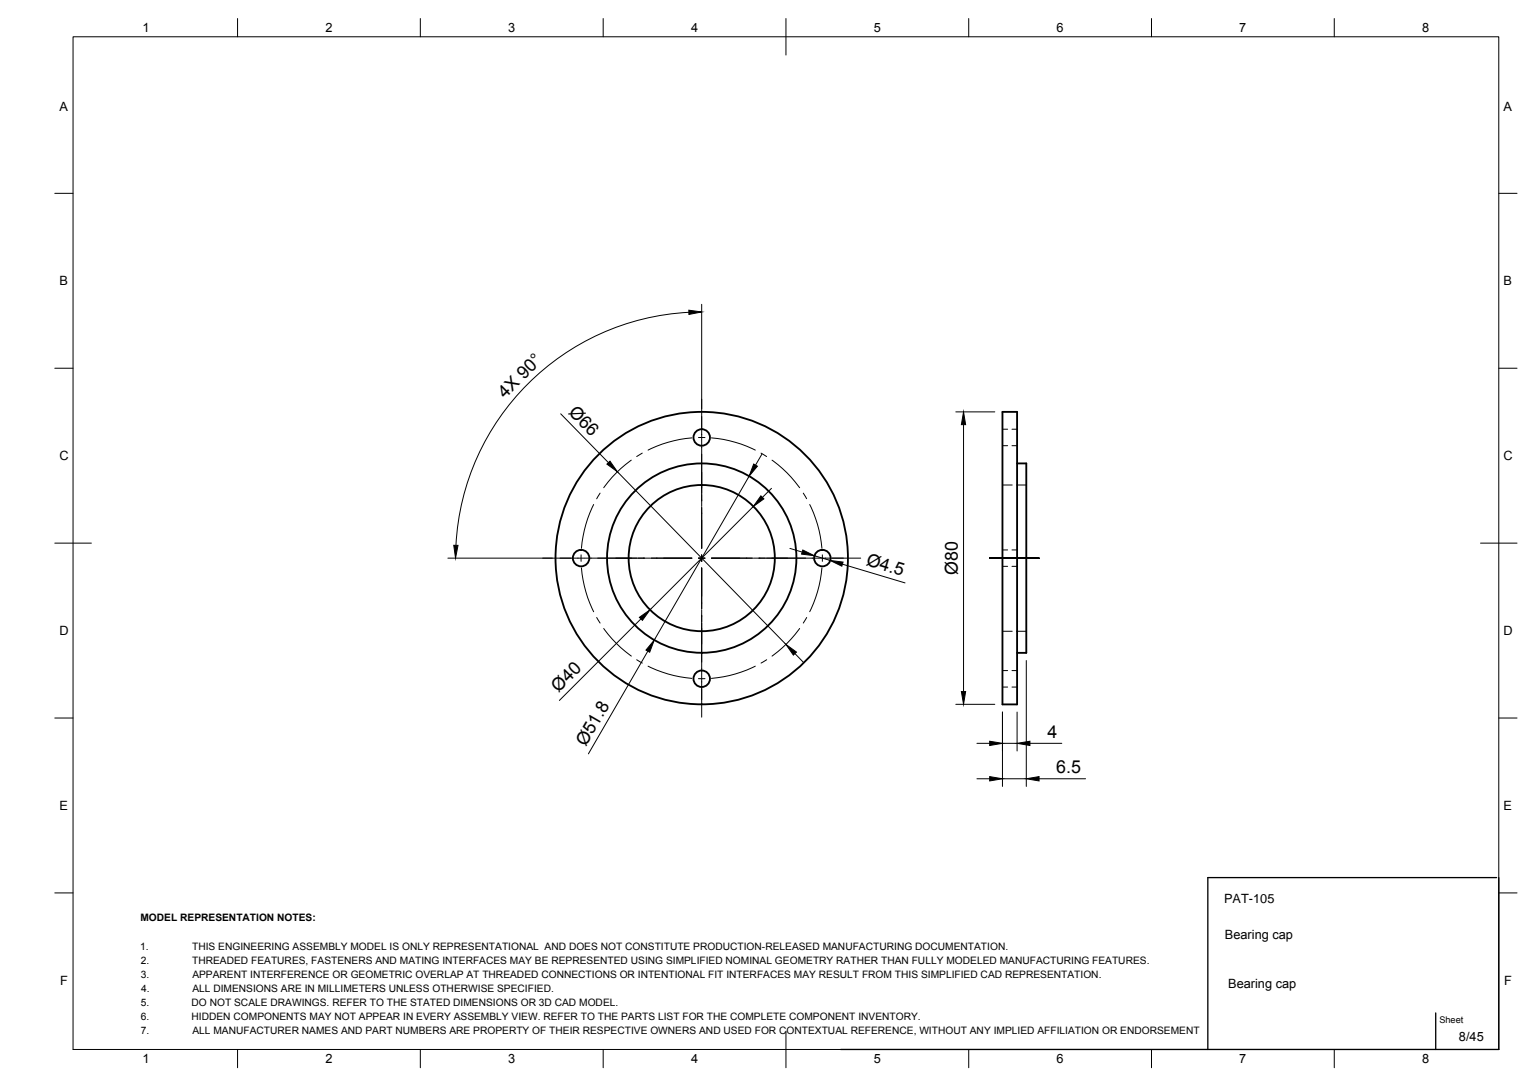
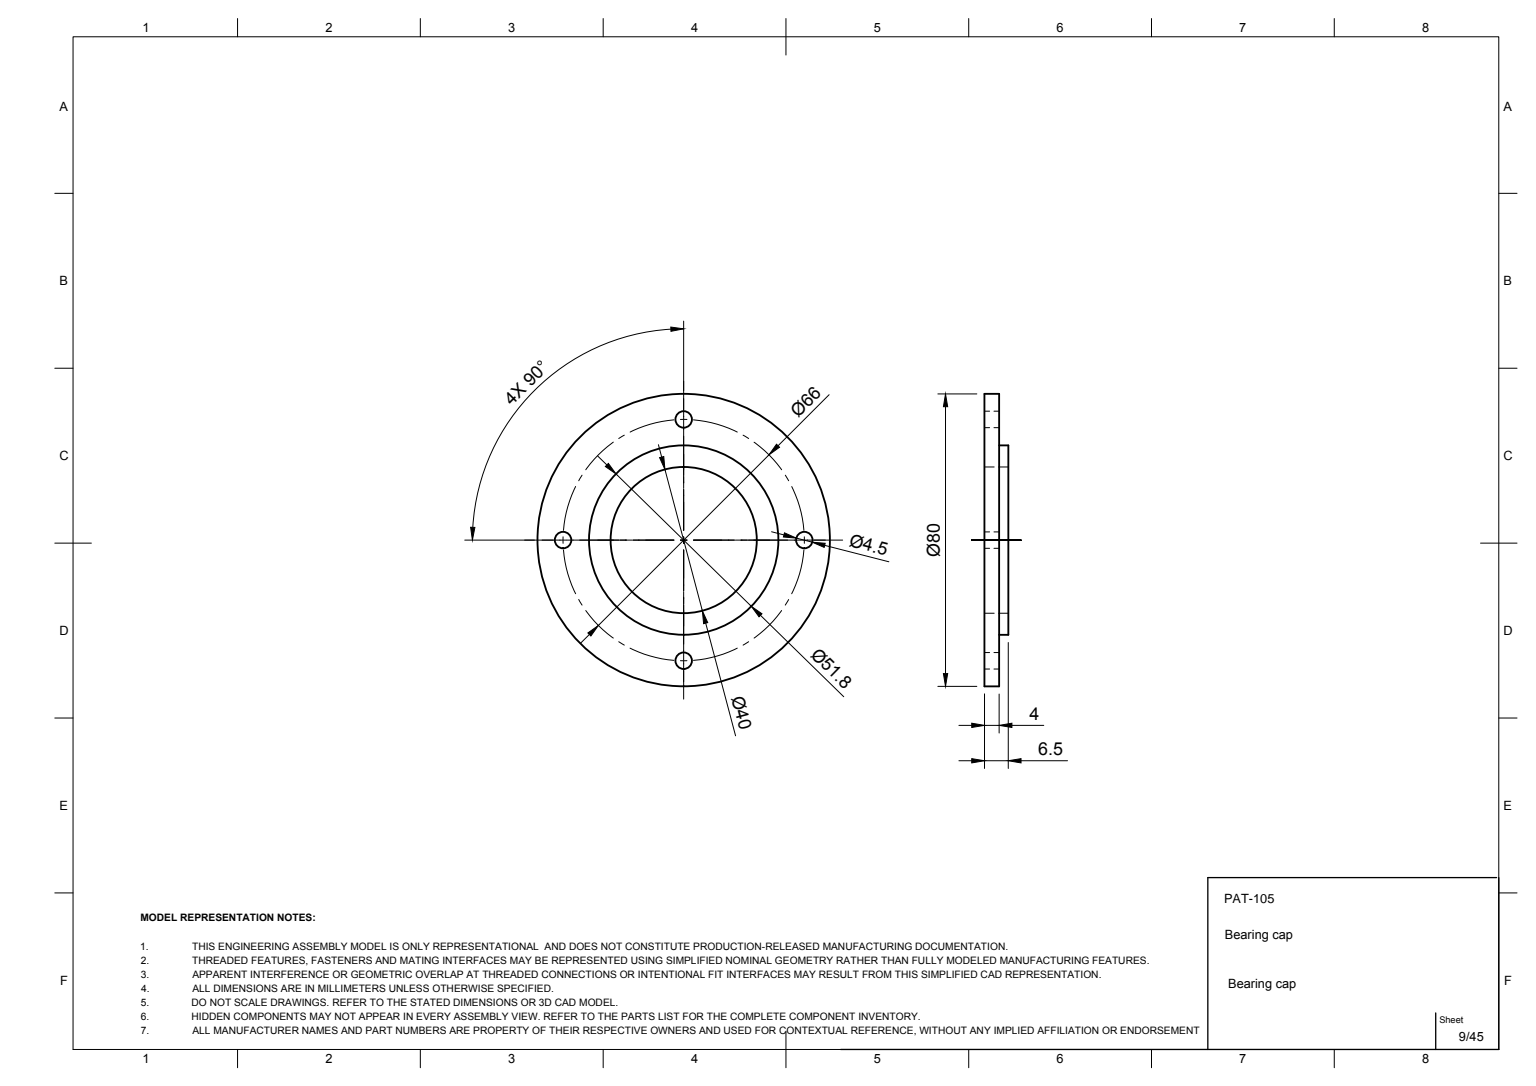
ISO-10303-21;
HEADER;
/* Generated by software containing ST-Developer
 * from STEP Tools, Inc. (www.steptools.com) 
 */

FILE_DESCRIPTION(
/* description */ ('Torque wrench calibration arm'),
/* implementation_level */ '2;1');

FILE_NAME(
/* name */ 'Bearing cap.step',
/* time_stamp */ '2026-10-28T03:24:52-07:00',
/* author */ (''),
/* organization */ (''),
/* preprocessor_version */ 'ST-DEVELOPER v20.2',
/* originating_system */ 'Autodesk Translation Framework v15.17.0.0',
/* authorisation */ '');

FILE_SCHEMA (('AUTOMOTIVE_DESIGN { 1 0 10303 214 3 1 1 }'));
ENDSEC;

DATA;
#10=MECHANICAL_DESIGN_GEOMETRIC_PRESENTATION_REPRESENTATION('',(#429),#12783);
#355=SHAPE_REPRESENTATION_RELATIONSHIP('SRR','None',#12936,#392);
#392=ADVANCED_BREP_SHAPE_REPRESENTATION('',(#483),#12745);
#429=STYLED_ITEM('',(#13212),#483);
#483=MANIFOLD_SOLID_BREP('Body1',#6498);
#561=FACE_BOUND('',#1374,.T.);
#562=FACE_BOUND('',#1378,.T.);
#563=FACE_BOUND('',#1379,.T.);
#564=FACE_BOUND('',#1380,.T.);
#565=FACE_BOUND('',#1381,.T.);
#566=FACE_BOUND('',#1382,.T.);
#567=FACE_BOUND('',#1384,.T.);
#568=FACE_BOUND('',#1385,.T.);
#569=FACE_BOUND('',#1386,.T.);
#570=FACE_BOUND('',#1387,.T.);
#571=FACE_BOUND('',#1388,.T.);
#692=PLANE('',#7109);
#693=PLANE('',#7116);
#694=PLANE('',#7117);
#943=FACE_OUTER_BOUND('',#1368,.T.);
#944=FACE_OUTER_BOUND('',#1369,.T.);
#945=FACE_OUTER_BOUND('',#1370,.T.);
#946=FACE_OUTER_BOUND('',#1371,.T.);
#947=FACE_OUTER_BOUND('',#1372,.T.);
#948=FACE_OUTER_BOUND('',#1373,.T.);
#949=FACE_OUTER_BOUND('',#1375,.T.);
#950=FACE_OUTER_BOUND('',#1376,.T.);
#951=FACE_OUTER_BOUND('',#1377,.T.);
#952=FACE_OUTER_BOUND('',#1383,.T.);
#1368=EDGE_LOOP('',(#4663,#4664,#4665,#4666));
#1369=EDGE_LOOP('',(#4667,#4668,#4669,#4670));
#1370=EDGE_LOOP('',(#4671,#4672,#4673,#4674));
#1371=EDGE_LOOP('',(#4675,#4676,#4677,#4678));
#1372=EDGE_LOOP('',(#4679,#4680,#4681,#4682));
#1373=EDGE_LOOP('',(#4683));
#1374=EDGE_LOOP('',(#4684));
#1375=EDGE_LOOP('',(#4685,#4686,#4687,#4688));
#1376=EDGE_LOOP('',(#4689,#4690,#4691,#4692));
#1377=EDGE_LOOP('',(#4693));
#1378=EDGE_LOOP('',(#4694));
#1379=EDGE_LOOP('',(#4695));
#1380=EDGE_LOOP('',(#4696));
#1381=EDGE_LOOP('',(#4697));
#1382=EDGE_LOOP('',(#4698));
#1383=EDGE_LOOP('',(#4699));
#1384=EDGE_LOOP('',(#4700));
#1385=EDGE_LOOP('',(#4701));
#1386=EDGE_LOOP('',(#4702));
#1387=EDGE_LOOP('',(#4703));
#1388=EDGE_LOOP('',(#4704));
#1882=LINE('',#10263,#2297);
#1883=LINE('',#10269,#2298);
#1884=LINE('',#10275,#2299);
#1885=LINE('',#10281,#2300);
#1886=LINE('',#10287,#2301);
#1887=LINE('',#10294,#2302);
#1888=LINE('',#10300,#2303);
#2297=VECTOR('',#8178,0.225);
#2298=VECTOR('',#8185,0.225);
#2299=VECTOR('',#8192,0.225);
#2300=VECTOR('',#8199,0.225);
#2301=VECTOR('',#8206,2.59);
#2302=VECTOR('',#8215,2.);
#2303=VECTOR('',#8222,4.);
#2676=CIRCLE('',#7095,0.225);
#2677=CIRCLE('',#7096,0.225);
#2678=CIRCLE('',#7098,0.225);
#2679=CIRCLE('',#7099,0.225);
#2680=CIRCLE('',#7101,0.225);
#2681=CIRCLE('',#7102,0.225);
#2682=CIRCLE('',#7104,0.225);
#2683=CIRCLE('',#7105,0.225);
#2684=CIRCLE('',#7107,2.59);
#2685=CIRCLE('',#7108,2.59);
#2686=CIRCLE('',#7110,2.);
#2687=CIRCLE('',#7112,2.);
#2688=CIRCLE('',#7114,4.);
#2689=CIRCLE('',#7115,4.);
#3075=VERTEX_POINT('',#10260);
#3076=VERTEX_POINT('',#10262);
#3077=VERTEX_POINT('',#10266);
#3078=VERTEX_POINT('',#10268);
#3079=VERTEX_POINT('',#10272);
#3080=VERTEX_POINT('',#10274);
#3081=VERTEX_POINT('',#10278);
#3082=VERTEX_POINT('',#10280);
#3083=VERTEX_POINT('',#10284);
#3084=VERTEX_POINT('',#10286);
#3085=VERTEX_POINT('',#10290);
#3086=VERTEX_POINT('',#10293);
#3087=VERTEX_POINT('',#10297);
#3088=VERTEX_POINT('',#10299);
#3689=EDGE_CURVE('',#3075,#3075,#2676,.T.);
#3690=EDGE_CURVE('',#3075,#3076,#1882,.T.);
#3691=EDGE_CURVE('',#3076,#3076,#2677,.T.);
#3692=EDGE_CURVE('',#3077,#3077,#2678,.T.);
#3693=EDGE_CURVE('',#3077,#3078,#1883,.T.);
#3694=EDGE_CURVE('',#3078,#3078,#2679,.T.);
#3695=EDGE_CURVE('',#3079,#3079,#2680,.T.);
#3696=EDGE_CURVE('',#3079,#3080,#1884,.T.);
#3697=EDGE_CURVE('',#3080,#3080,#2681,.T.);
#3698=EDGE_CURVE('',#3081,#3081,#2682,.T.);
#3699=EDGE_CURVE('',#3081,#3082,#1885,.T.);
#3700=EDGE_CURVE('',#3082,#3082,#2683,.T.);
#3701=EDGE_CURVE('',#3083,#3083,#2684,.T.);
#3702=EDGE_CURVE('',#3083,#3084,#1886,.T.);
#3703=EDGE_CURVE('',#3084,#3084,#2685,.T.);
#3704=EDGE_CURVE('',#3085,#3085,#2686,.T.);
#3705=EDGE_CURVE('',#3085,#3086,#1887,.T.);
#3706=EDGE_CURVE('',#3086,#3086,#2687,.T.);
#3707=EDGE_CURVE('',#3087,#3087,#2688,.T.);
#3708=EDGE_CURVE('',#3087,#3088,#1888,.T.);
#3709=EDGE_CURVE('',#3088,#3088,#2689,.T.);
#4663=ORIENTED_EDGE('',*,*,#3689,.F.);
#4664=ORIENTED_EDGE('',*,*,#3690,.T.);
#4665=ORIENTED_EDGE('',*,*,#3691,.F.);
#4666=ORIENTED_EDGE('',*,*,#3690,.F.);
#4667=ORIENTED_EDGE('',*,*,#3692,.F.);
#4668=ORIENTED_EDGE('',*,*,#3693,.T.);
#4669=ORIENTED_EDGE('',*,*,#3694,.F.);
#4670=ORIENTED_EDGE('',*,*,#3693,.F.);
#4671=ORIENTED_EDGE('',*,*,#3695,.F.);
#4672=ORIENTED_EDGE('',*,*,#3696,.T.);
#4673=ORIENTED_EDGE('',*,*,#3697,.F.);
#4674=ORIENTED_EDGE('',*,*,#3696,.F.);
#4675=ORIENTED_EDGE('',*,*,#3698,.F.);
#4676=ORIENTED_EDGE('',*,*,#3699,.T.);
#4677=ORIENTED_EDGE('',*,*,#3700,.F.);
#4678=ORIENTED_EDGE('',*,*,#3699,.F.);
#4679=ORIENTED_EDGE('',*,*,#3701,.F.);
#4680=ORIENTED_EDGE('',*,*,#3702,.T.);
#4681=ORIENTED_EDGE('',*,*,#3703,.F.);
#4682=ORIENTED_EDGE('',*,*,#3702,.F.);
#4683=ORIENTED_EDGE('',*,*,#3701,.T.);
#4684=ORIENTED_EDGE('',*,*,#3704,.T.);
#4685=ORIENTED_EDGE('',*,*,#3704,.F.);
#4686=ORIENTED_EDGE('',*,*,#3705,.T.);
#4687=ORIENTED_EDGE('',*,*,#3706,.T.);
#4688=ORIENTED_EDGE('',*,*,#3705,.F.);
#4689=ORIENTED_EDGE('',*,*,#3707,.F.);
#4690=ORIENTED_EDGE('',*,*,#3708,.T.);
#4691=ORIENTED_EDGE('',*,*,#3709,.T.);
#4692=ORIENTED_EDGE('',*,*,#3708,.F.);
#4693=ORIENTED_EDGE('',*,*,#3707,.T.);
#4694=ORIENTED_EDGE('',*,*,#3703,.T.);
#4695=ORIENTED_EDGE('',*,*,#3700,.T.);
#4696=ORIENTED_EDGE('',*,*,#3697,.T.);
#4697=ORIENTED_EDGE('',*,*,#3694,.T.);
#4698=ORIENTED_EDGE('',*,*,#3691,.T.);
#4699=ORIENTED_EDGE('',*,*,#3709,.F.);
#4700=ORIENTED_EDGE('',*,*,#3706,.F.);
#4701=ORIENTED_EDGE('',*,*,#3698,.T.);
#4702=ORIENTED_EDGE('',*,*,#3695,.T.);
#4703=ORIENTED_EDGE('',*,*,#3692,.T.);
#4704=ORIENTED_EDGE('',*,*,#3689,.T.);
#6015=CYLINDRICAL_SURFACE('',#7094,0.225);
#6016=CYLINDRICAL_SURFACE('',#7097,0.225);
#6017=CYLINDRICAL_SURFACE('',#7100,0.225);
#6018=CYLINDRICAL_SURFACE('',#7103,0.225);
#6019=CYLINDRICAL_SURFACE('',#7106,2.59);
#6020=CYLINDRICAL_SURFACE('',#7111,2.);
#6021=CYLINDRICAL_SURFACE('',#7113,4.);
#6168=ADVANCED_FACE('',(#943),#6015,.F.);
#6169=ADVANCED_FACE('',(#944),#6016,.F.);
#6170=ADVANCED_FACE('',(#945),#6017,.F.);
#6171=ADVANCED_FACE('',(#946),#6018,.F.);
#6172=ADVANCED_FACE('',(#947),#6019,.T.);
#6173=ADVANCED_FACE('',(#948,#561),#692,.T.);
#6174=ADVANCED_FACE('',(#949),#6020,.F.);
#6175=ADVANCED_FACE('',(#950),#6021,.T.);
#6176=ADVANCED_FACE('',(#951,#562,#563,#564,#565,#566),#693,.T.);
#6177=ADVANCED_FACE('',(#952,#567,#568,#569,#570,#571),#694,.F.);
#6498=CLOSED_SHELL('',(#6168,#6169,#6170,#6171,#6172,#6173,#6174,#6175,
#6176,#6177));
#7093=AXIS2_PLACEMENT_3D('',#10258,#8172,#8173);
#7094=AXIS2_PLACEMENT_3D('',#10259,#8174,#8175);
#7095=AXIS2_PLACEMENT_3D('',#10261,#8176,#8177);
#7096=AXIS2_PLACEMENT_3D('',#10264,#8179,#8180);
#7097=AXIS2_PLACEMENT_3D('',#10265,#8181,#8182);
#7098=AXIS2_PLACEMENT_3D('',#10267,#8183,#8184);
#7099=AXIS2_PLACEMENT_3D('',#10270,#8186,#8187);
#7100=AXIS2_PLACEMENT_3D('',#10271,#8188,#8189);
#7101=AXIS2_PLACEMENT_3D('',#10273,#8190,#8191);
#7102=AXIS2_PLACEMENT_3D('',#10276,#8193,#8194);
#7103=AXIS2_PLACEMENT_3D('',#10277,#8195,#8196);
#7104=AXIS2_PLACEMENT_3D('',#10279,#8197,#8198);
#7105=AXIS2_PLACEMENT_3D('',#10282,#8200,#8201);
#7106=AXIS2_PLACEMENT_3D('',#10283,#8202,#8203);
#7107=AXIS2_PLACEMENT_3D('',#10285,#8204,#8205);
#7108=AXIS2_PLACEMENT_3D('',#10288,#8207,#8208);
#7109=AXIS2_PLACEMENT_3D('',#10289,#8209,#8210);
#7110=AXIS2_PLACEMENT_3D('',#10291,#8211,#8212);
#7111=AXIS2_PLACEMENT_3D('',#10292,#8213,#8214);
#7112=AXIS2_PLACEMENT_3D('',#10295,#8216,#8217);
#7113=AXIS2_PLACEMENT_3D('',#10296,#8218,#8219);
#7114=AXIS2_PLACEMENT_3D('',#10298,#8220,#8221);
#7115=AXIS2_PLACEMENT_3D('',#10301,#8223,#8224);
#7116=AXIS2_PLACEMENT_3D('',#10302,#8225,#8226);
#7117=AXIS2_PLACEMENT_3D('',#10303,#8227,#8228);
#8172=DIRECTION('axis',(0.,0.,1.));
#8173=DIRECTION('refdir',(1.,0.,0.));
#8174=DIRECTION('center_axis',(0.,1.,0.));
#8175=DIRECTION('ref_axis',(1.,0.,0.));
#8176=DIRECTION('center_axis',(0.,1.,0.));
#8177=DIRECTION('ref_axis',(1.,0.,0.));
#8178=DIRECTION('',(0.,1.,0.));
#8179=DIRECTION('center_axis',(0.,-1.,0.));
#8180=DIRECTION('ref_axis',(1.,0.,0.));
#8181=DIRECTION('center_axis',(0.,1.,0.));
#8182=DIRECTION('ref_axis',(1.,0.,0.));
#8183=DIRECTION('center_axis',(0.,1.,0.));
#8184=DIRECTION('ref_axis',(1.,0.,0.));
#8185=DIRECTION('',(0.,1.,0.));
#8186=DIRECTION('center_axis',(0.,-1.,0.));
#8187=DIRECTION('ref_axis',(1.,0.,0.));
#8188=DIRECTION('center_axis',(0.,1.,0.));
#8189=DIRECTION('ref_axis',(1.,0.,0.));
#8190=DIRECTION('center_axis',(0.,1.,0.));
#8191=DIRECTION('ref_axis',(1.,0.,0.));
#8192=DIRECTION('',(0.,1.,0.));
#8193=DIRECTION('center_axis',(0.,-1.,0.));
#8194=DIRECTION('ref_axis',(1.,0.,0.));
#8195=DIRECTION('center_axis',(0.,1.,0.));
#8196=DIRECTION('ref_axis',(1.,0.,0.));
#8197=DIRECTION('center_axis',(0.,1.,0.));
#8198=DIRECTION('ref_axis',(1.,0.,0.));
#8199=DIRECTION('',(0.,1.,0.));
#8200=DIRECTION('center_axis',(0.,-1.,0.));
#8201=DIRECTION('ref_axis',(1.,0.,0.));
#8202=DIRECTION('center_axis',(0.,1.,0.));
#8203=DIRECTION('ref_axis',(1.,0.,0.));
#8204=DIRECTION('center_axis',(0.,1.,0.));
#8205=DIRECTION('ref_axis',(1.,0.,0.));
#8206=DIRECTION('',(0.,-1.,0.));
#8207=DIRECTION('center_axis',(0.,-1.,0.));
#8208=DIRECTION('ref_axis',(1.,0.,0.));
#8209=DIRECTION('center_axis',(0.,1.,0.));
#8210=DIRECTION('ref_axis',(1.,0.,0.));
#8211=DIRECTION('center_axis',(0.,-1.,0.));
#8212=DIRECTION('ref_axis',(1.,0.,0.));
#8213=DIRECTION('center_axis',(0.,1.,0.));
#8214=DIRECTION('ref_axis',(1.,0.,0.));
#8215=DIRECTION('',(0.,-1.,0.));
#8216=DIRECTION('center_axis',(0.,-1.,0.));
#8217=DIRECTION('ref_axis',(1.,0.,0.));
#8218=DIRECTION('center_axis',(0.,1.,0.));
#8219=DIRECTION('ref_axis',(1.,0.,0.));
#8220=DIRECTION('center_axis',(0.,1.,0.));
#8221=DIRECTION('ref_axis',(1.,0.,0.));
#8222=DIRECTION('',(0.,-1.,0.));
#8223=DIRECTION('center_axis',(0.,1.,0.));
#8224=DIRECTION('ref_axis',(1.,0.,0.));
#8225=DIRECTION('center_axis',(0.,1.,0.));
#8226=DIRECTION('ref_axis',(1.,0.,0.));
#8227=DIRECTION('center_axis',(0.,1.,0.));
#8228=DIRECTION('ref_axis',(1.,0.,0.));
#10258=CARTESIAN_POINT('',(0.,0.,0.));
#10259=CARTESIAN_POINT('Origin',(-3.3,-0.5,8.));
#10260=CARTESIAN_POINT('',(-3.525,-0.4,8.));
#10261=CARTESIAN_POINT('Origin',(-3.3,-0.4,8.));
#10262=CARTESIAN_POINT('',(-3.525,0.,8.));
#10263=CARTESIAN_POINT('',(-3.525,-0.5,8.));
#10264=CARTESIAN_POINT('Origin',(-3.3,0.,8.));
#10265=CARTESIAN_POINT('Origin',(2.02066721859313E-16,-0.5,11.3));
#10266=CARTESIAN_POINT('',(-0.225,-0.4,11.3));
#10267=CARTESIAN_POINT('Origin',(2.02066721859313E-16,-0.4,11.3));
#10268=CARTESIAN_POINT('',(-0.225,0.,11.3));
#10269=CARTESIAN_POINT('',(-0.225,-0.5,11.3));
#10270=CARTESIAN_POINT('Origin',(2.02066721859313E-16,0.,11.3));
#10271=CARTESIAN_POINT('Origin',(3.3,-0.5,8.));
#10272=CARTESIAN_POINT('',(3.075,-0.4,8.));
#10273=CARTESIAN_POINT('Origin',(3.3,-0.4,8.));
#10274=CARTESIAN_POINT('',(3.075,0.,8.));
#10275=CARTESIAN_POINT('',(3.075,-0.5,8.));
#10276=CARTESIAN_POINT('Origin',(3.3,0.,8.));
#10277=CARTESIAN_POINT('Origin',(-6.0620016557794E-16,-0.5,4.7));
#10278=CARTESIAN_POINT('',(-0.225000000000001,-0.4,4.7));
#10279=CARTESIAN_POINT('Origin',(-6.0620016557794E-16,-0.4,4.7));
#10280=CARTESIAN_POINT('',(-0.225000000000001,0.,4.7));
#10281=CARTESIAN_POINT('',(-0.225000000000001,-0.5,4.7));
#10282=CARTESIAN_POINT('Origin',(-6.0620016557794E-16,0.,4.7));
#10283=CARTESIAN_POINT('Origin',(0.,0.,8.));
#10284=CARTESIAN_POINT('',(-2.59,0.25,8.));
#10285=CARTESIAN_POINT('Origin',(0.,0.25,8.));
#10286=CARTESIAN_POINT('',(-2.59,0.,8.));
#10287=CARTESIAN_POINT('',(-2.59,0.,8.));
#10288=CARTESIAN_POINT('Origin',(0.,0.,8.));
#10289=CARTESIAN_POINT('Origin',(0.,0.25,8.));
#10290=CARTESIAN_POINT('',(-2.,0.25,8.));
#10291=CARTESIAN_POINT('Origin',(0.,0.25,8.));
#10292=CARTESIAN_POINT('Origin',(0.,-0.4,8.));
#10293=CARTESIAN_POINT('',(-2.,-0.4,8.));
#10294=CARTESIAN_POINT('',(-2.,-0.4,8.));
#10295=CARTESIAN_POINT('Origin',(0.,-0.4,8.));
#10296=CARTESIAN_POINT('Origin',(0.,-0.4,8.));
#10297=CARTESIAN_POINT('',(-4.,0.,8.));
#10298=CARTESIAN_POINT('Origin',(0.,0.,8.));
#10299=CARTESIAN_POINT('',(-4.,-0.4,8.));
#10300=CARTESIAN_POINT('',(-4.,-0.4,8.));
#10301=CARTESIAN_POINT('Origin',(0.,-0.4,8.));
#10302=CARTESIAN_POINT('Origin',(0.,0.,8.));
#10303=CARTESIAN_POINT('Origin',(0.,-0.4,8.));
#12701=UNCERTAINTY_MEASURE_WITH_UNIT(LENGTH_MEASURE(0.001),#12784,
'DISTANCE_ACCURACY_VALUE',
'Maximum model space distance between geometric entities at asserted c
onnectivities');
#12739=UNCERTAINTY_MEASURE_WITH_UNIT(LENGTH_MEASURE(0.001),#12784,
'DISTANCE_ACCURACY_VALUE',
'Maximum model space distance between geometric entities at asserted c
onnectivities');
#12745=(
GEOMETRIC_REPRESENTATION_CONTEXT(3)
GLOBAL_UNCERTAINTY_ASSIGNED_CONTEXT((#12701))
GLOBAL_UNIT_ASSIGNED_CONTEXT((#12784,#12786,#12787))
REPRESENTATION_CONTEXT('','3D')
);
#12783=(
GEOMETRIC_REPRESENTATION_CONTEXT(3)
GLOBAL_UNCERTAINTY_ASSIGNED_CONTEXT((#12739))
GLOBAL_UNIT_ASSIGNED_CONTEXT((#12784,#12786,#12787))
REPRESENTATION_CONTEXT('','3D')
);
#12784=(
LENGTH_UNIT()
NAMED_UNIT(*)
SI_UNIT(.CENTI.,.METRE.)
);
#12786=(
NAMED_UNIT(*)
PLANE_ANGLE_UNIT()
SI_UNIT($,.RADIAN.)
);
#12787=(
NAMED_UNIT(*)
SI_UNIT($,.STERADIAN.)
SOLID_ANGLE_UNIT()
);
#12793=SHAPE_DEFINITION_REPRESENTATION(#12836,#12936);
#12836=PRODUCT_DEFINITION_SHAPE('',$,#12980);
#12936=SHAPE_REPRESENTATION('',(#7093),#12745);
#12974=PRODUCT_DEFINITION_CONTEXT('part definition',#13105,'design');
#12980=PRODUCT_DEFINITION('Bearing cap','Bearing cap',#13023,#12974);
#13023=PRODUCT_DEFINITION_FORMATION('',$,#13112);
#13105=APPLICATION_CONTEXT(
'Core Data for Automotive Mechanical Design Process');
#13106=PRODUCT_CONTEXT('part definition',#13105,'mechanical');
#13112=PRODUCT('Bearing cap','Bearing cap','Bearing cap',(#13106));
#13206=COLOUR_RGB('Grey',0.48,0.52,0.57);
#13207=FILL_AREA_STYLE_COLOUR('',#13206);
#13208=FILL_AREA_STYLE('',(#13207));
#13209=SURFACE_STYLE_FILL_AREA(#13208);
#13210=SURFACE_SIDE_STYLE('',(#13209));
#13211=SURFACE_STYLE_USAGE(.BOTH.,#13210);
#13212=PRESENTATION_STYLE_ASSIGNMENT((#13211));
ENDSEC;
END-ISO-10303-21;
